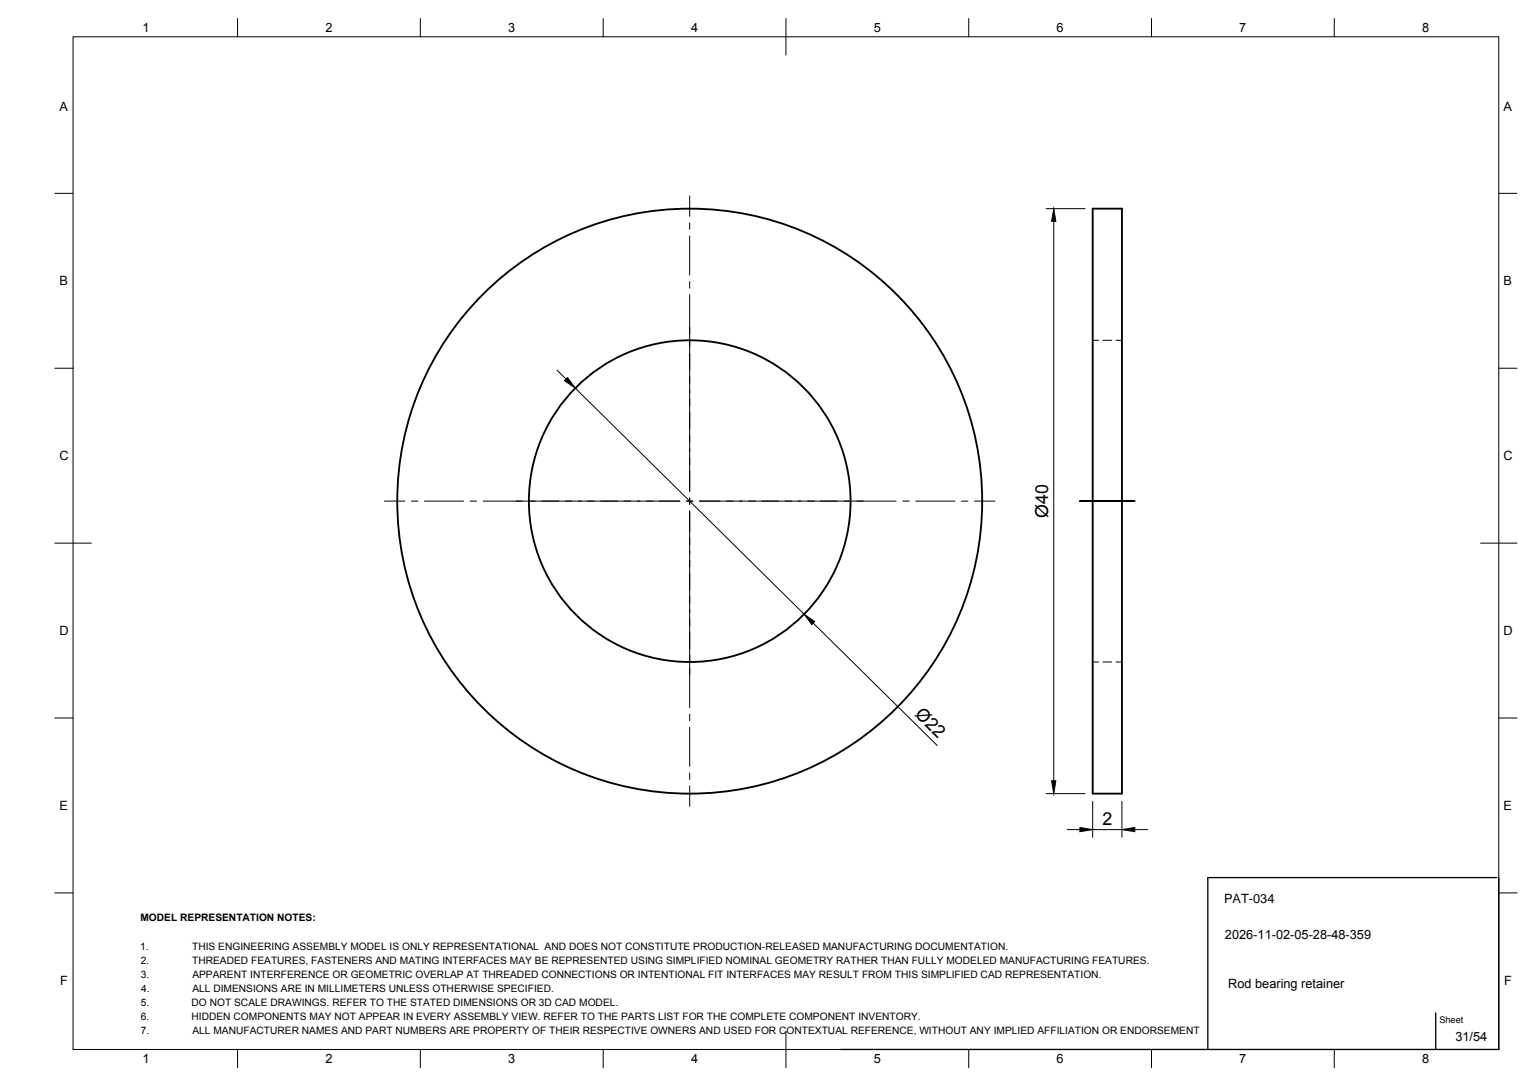
ISO-10303-21;
HEADER;
/* Generated by software containing ST-Developer
 * from STEP Tools, Inc. (www.steptools.com) 
 */

FILE_DESCRIPTION(
/* description */ ('Fatigue rig crank-slider'),
/* implementation_level */ '2;1');

FILE_NAME(
/* name */ 'Rod bearing retainer.step',
/* time_stamp */ '2026-10-28T03:24:50-07:00',
/* author */ (''),
/* organization */ (''),
/* preprocessor_version */ 'ST-DEVELOPER v20.2',
/* originating_system */ 'Autodesk Translation Framework v15.17.0.0',
/* authorisation */ '');

FILE_SCHEMA (('AUTOMOTIVE_DESIGN { 1 0 10303 214 3 1 1 }'));
ENDSEC;

DATA;
#10=MECHANICAL_DESIGN_GEOMETRIC_PRESENTATION_REPRESENTATION('',(#616),#16911);
#515=SHAPE_REPRESENTATION_RELATIONSHIP('SRR','None',#17157,#565);
#565=ADVANCED_BREP_SHAPE_REPRESENTATION('',(#673),#16886);
#616=STYLED_ITEM('',(#17487),#673);
#673=MANIFOLD_SOLID_BREP('Body1',#8909);
#846=FACE_BOUND('',#2198,.T.);
#847=FACE_BOUND('',#2200,.T.);
#1086=PLANE('',#10077);
#1087=PLANE('',#10078);
#1526=FACE_OUTER_BOUND('',#2195,.T.);
#1527=FACE_OUTER_BOUND('',#2196,.T.);
#1528=FACE_OUTER_BOUND('',#2197,.T.);
#1529=FACE_OUTER_BOUND('',#2199,.T.);
#2195=EDGE_LOOP('',(#7292,#7293,#7294,#7295));
#2196=EDGE_LOOP('',(#7296,#7297,#7298,#7299));
#2197=EDGE_LOOP('',(#7300));
#2198=EDGE_LOOP('',(#7301));
#2199=EDGE_LOOP('',(#7302));
#2200=EDGE_LOOP('',(#7303));
#2839=LINE('',#15373,#3485);
#2840=LINE('',#15379,#3486);
#3485=VECTOR('',#12105,1.1);
#3486=VECTOR('',#12112,2.);
#3985=CIRCLE('',#10072,1.1);
#3986=CIRCLE('',#10073,1.1);
#3987=CIRCLE('',#10075,2.);
#3988=CIRCLE('',#10076,2.);
#4589=VERTEX_POINT('',#15370);
#4590=VERTEX_POINT('',#15372);
#4591=VERTEX_POINT('',#15376);
#4592=VERTEX_POINT('',#15378);
#5544=EDGE_CURVE('',#4589,#4589,#3985,.T.);
#5545=EDGE_CURVE('',#4589,#4590,#2839,.T.);
#5546=EDGE_CURVE('',#4590,#4590,#3986,.T.);
#5547=EDGE_CURVE('',#4591,#4591,#3987,.T.);
#5548=EDGE_CURVE('',#4591,#4592,#2840,.T.);
#5549=EDGE_CURVE('',#4592,#4592,#3988,.T.);
#7292=ORIENTED_EDGE('',*,*,#5544,.F.);
#7293=ORIENTED_EDGE('',*,*,#5545,.T.);
#7294=ORIENTED_EDGE('',*,*,#5546,.T.);
#7295=ORIENTED_EDGE('',*,*,#5545,.F.);
#7296=ORIENTED_EDGE('',*,*,#5547,.F.);
#7297=ORIENTED_EDGE('',*,*,#5548,.T.);
#7298=ORIENTED_EDGE('',*,*,#5549,.T.);
#7299=ORIENTED_EDGE('',*,*,#5548,.F.);
#7300=ORIENTED_EDGE('',*,*,#5547,.T.);
#7301=ORIENTED_EDGE('',*,*,#5544,.T.);
#7302=ORIENTED_EDGE('',*,*,#5549,.F.);
#7303=ORIENTED_EDGE('',*,*,#5546,.F.);
#8305=CYLINDRICAL_SURFACE('',#10071,1.1);
#8306=CYLINDRICAL_SURFACE('',#10074,2.);
#8664=ADVANCED_FACE('',(#1526),#8305,.F.);
#8665=ADVANCED_FACE('',(#1527),#8306,.T.);
#8666=ADVANCED_FACE('',(#1528,#846),#1086,.T.);
#8667=ADVANCED_FACE('',(#1529,#847),#1087,.F.);
#8909=CLOSED_SHELL('',(#8664,#8665,#8666,#8667));
#10070=AXIS2_PLACEMENT_3D('',#15368,#12099,#12100);
#10071=AXIS2_PLACEMENT_3D('',#15369,#12101,#12102);
#10072=AXIS2_PLACEMENT_3D('',#15371,#12103,#12104);
#10073=AXIS2_PLACEMENT_3D('',#15374,#12106,#12107);
#10074=AXIS2_PLACEMENT_3D('',#15375,#12108,#12109);
#10075=AXIS2_PLACEMENT_3D('',#15377,#12110,#12111);
#10076=AXIS2_PLACEMENT_3D('',#15380,#12113,#12114);
#10077=AXIS2_PLACEMENT_3D('',#15381,#12115,#12116);
#10078=AXIS2_PLACEMENT_3D('',#15382,#12117,#12118);
#12099=DIRECTION('axis',(0.,0.,1.));
#12100=DIRECTION('refdir',(1.,0.,0.));
#12101=DIRECTION('center_axis',(0.,1.,0.));
#12102=DIRECTION('ref_axis',(1.,0.,0.));
#12103=DIRECTION('center_axis',(0.,-1.,0.));
#12104=DIRECTION('ref_axis',(1.,0.,0.));
#12105=DIRECTION('',(0.,-1.,0.));
#12106=DIRECTION('center_axis',(0.,-1.,0.));
#12107=DIRECTION('ref_axis',(1.,0.,0.));
#12108=DIRECTION('center_axis',(0.,1.,0.));
#12109=DIRECTION('ref_axis',(1.,0.,0.));
#12110=DIRECTION('center_axis',(0.,1.,0.));
#12111=DIRECTION('ref_axis',(1.,0.,0.));
#12112=DIRECTION('',(0.,-1.,0.));
#12113=DIRECTION('center_axis',(0.,1.,0.));
#12114=DIRECTION('ref_axis',(1.,0.,0.));
#12115=DIRECTION('center_axis',(0.,1.,0.));
#12116=DIRECTION('ref_axis',(1.,0.,0.));
#12117=DIRECTION('center_axis',(0.,1.,0.));
#12118=DIRECTION('ref_axis',(1.,0.,0.));
#15368=CARTESIAN_POINT('',(0.,0.,0.));
#15369=CARTESIAN_POINT('Origin',(1.,3.3,12.));
#15370=CARTESIAN_POINT('',(-0.1,3.5,12.));
#15371=CARTESIAN_POINT('Origin',(1.,3.5,12.));
#15372=CARTESIAN_POINT('',(-0.1,3.3,12.));
#15373=CARTESIAN_POINT('',(-0.1,3.3,12.));
#15374=CARTESIAN_POINT('Origin',(1.,3.3,12.));
#15375=CARTESIAN_POINT('Origin',(1.,3.3,12.));
#15376=CARTESIAN_POINT('',(-1.,3.5,12.));
#15377=CARTESIAN_POINT('Origin',(1.,3.5,12.));
#15378=CARTESIAN_POINT('',(-1.,3.3,12.));
#15379=CARTESIAN_POINT('',(-1.,3.3,12.));
#15380=CARTESIAN_POINT('Origin',(1.,3.3,12.));
#15381=CARTESIAN_POINT('Origin',(1.,3.5,12.));
#15382=CARTESIAN_POINT('Origin',(1.,3.3,12.));
#16827=UNCERTAINTY_MEASURE_WITH_UNIT(LENGTH_MEASURE(0.001),#16912,
'DISTANCE_ACCURACY_VALUE',
'Maximum model space distance between geometric entities at asserted c
onnectivities');
#16852=UNCERTAINTY_MEASURE_WITH_UNIT(LENGTH_MEASURE(0.001),#16912,
'DISTANCE_ACCURACY_VALUE',
'Maximum model space distance between geometric entities at asserted c
onnectivities');
#16886=(
GEOMETRIC_REPRESENTATION_CONTEXT(3)
GLOBAL_UNCERTAINTY_ASSIGNED_CONTEXT((#16827))
GLOBAL_UNIT_ASSIGNED_CONTEXT((#16912,#16914,#16915))
REPRESENTATION_CONTEXT('','3D')
);
#16911=(
GEOMETRIC_REPRESENTATION_CONTEXT(3)
GLOBAL_UNCERTAINTY_ASSIGNED_CONTEXT((#16852))
GLOBAL_UNIT_ASSIGNED_CONTEXT((#16912,#16914,#16915))
REPRESENTATION_CONTEXT('','3D')
);
#16912=(
LENGTH_UNIT()
NAMED_UNIT(*)
SI_UNIT(.CENTI.,.METRE.)
);
#16914=(
NAMED_UNIT(*)
PLANE_ANGLE_UNIT()
SI_UNIT($,.RADIAN.)
);
#16915=(
NAMED_UNIT(*)
SI_UNIT($,.STERADIAN.)
SOLID_ANGLE_UNIT()
);
#16949=SHAPE_DEFINITION_REPRESENTATION(#17009,#17157);
#17009=PRODUCT_DEFINITION_SHAPE('',$,#17216);
#17157=SHAPE_REPRESENTATION('',(#10070),#16886);
#17182=PRODUCT_DEFINITION_CONTEXT('part definition',#17358,'design');
#17216=PRODUCT_DEFINITION('Rod bearing retainer','Rod bearing retainer',
#17274,#17182);
#17274=PRODUCT_DEFINITION_FORMATION('',$,#17393);
#17358=APPLICATION_CONTEXT(
'Core Data for Automotive Mechanical Design Process');
#17359=PRODUCT_CONTEXT('part definition',#17358,'mechanical');
#17393=PRODUCT('Rod bearing retainer','Rod bearing retainer',
'Rod bearing retainer',(#17359));
#17481=COLOUR_RGB('Grey',0.48,0.52,0.57);
#17482=FILL_AREA_STYLE_COLOUR('',#17481);
#17483=FILL_AREA_STYLE('',(#17482));
#17484=SURFACE_STYLE_FILL_AREA(#17483);
#17485=SURFACE_SIDE_STYLE('',(#17484));
#17486=SURFACE_STYLE_USAGE(.BOTH.,#17485);
#17487=PRESENTATION_STYLE_ASSIGNMENT((#17486));
ENDSEC;
END-ISO-10303-21;
